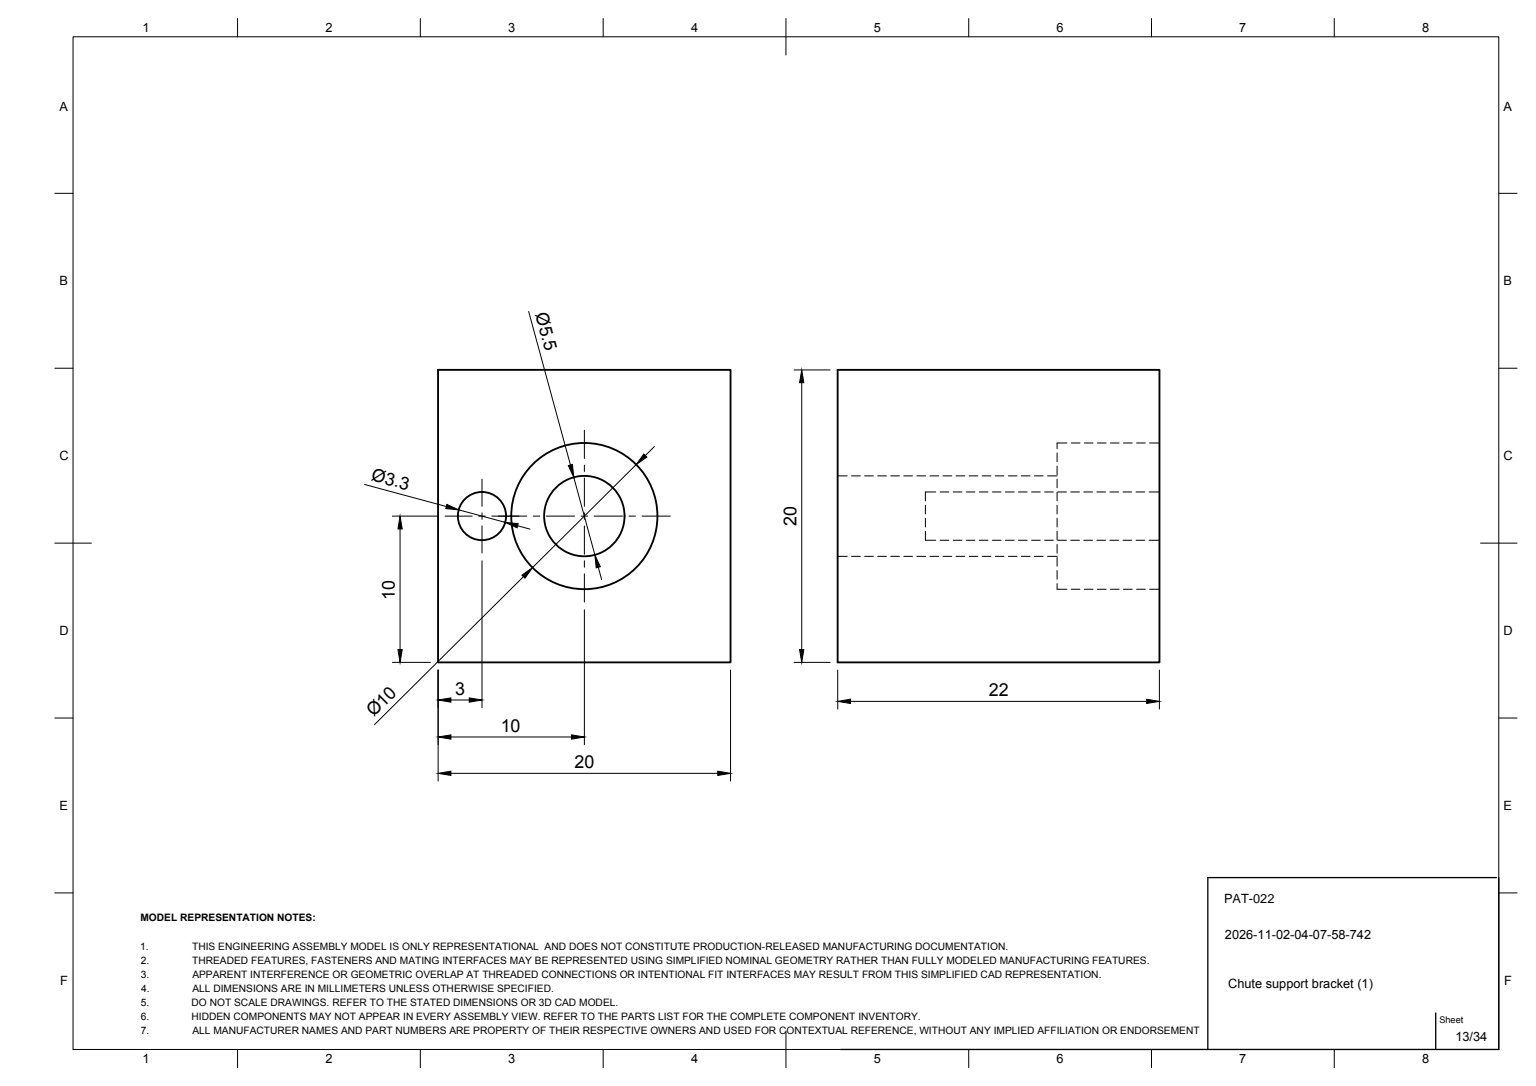
ISO-10303-21;
HEADER;
/* Generated by software containing ST-Developer
 * from STEP Tools, Inc. (www.steptools.com) 
 */

FILE_DESCRIPTION(
/* description */ ('Chute with adjustable gate'),
/* implementation_level */ '2;1');

FILE_NAME(
/* name */ 'Chute support bracket (1).step',
/* time_stamp */ '2026-10-27T10:52:28-07:00',
/* author */ (''),
/* organization */ (''),
/* preprocessor_version */ 'ST-DEVELOPER v20.2',
/* originating_system */ 'Autodesk Translation Framework v15.17.0.0',
/* authorisation */ '');

FILE_SCHEMA (('AUTOMOTIVE_DESIGN { 1 0 10303 214 3 1 1 }'));
ENDSEC;

DATA;
#10=MECHANICAL_DESIGN_GEOMETRIC_PRESENTATION_REPRESENTATION('',(#422),#13094);
#358=SHAPE_REPRESENTATION_RELATIONSHIP('SRR','None',#13259,#390);
#390=ADVANCED_BREP_SHAPE_REPRESENTATION('',(#454),#13068);
#422=STYLED_ITEM('',(#13474),#454);
#454=MANIFOLD_SOLID_BREP('Body1',#7605);
#504=FACE_BOUND('',#1432,.T.);
#505=FACE_BOUND('',#1435,.T.);
#506=FACE_BOUND('',#1438,.T.);
#507=FACE_BOUND('',#1439,.T.);
#644=PLANE('',#8099);
#645=PLANE('',#8103);
#646=PLANE('',#8107);
#647=PLANE('',#8108);
#648=PLANE('',#8109);
#649=PLANE('',#8110);
#650=PLANE('',#8111);
#651=PLANE('',#8112);
#983=FACE_OUTER_BOUND('',#1428,.T.);
#984=FACE_OUTER_BOUND('',#1429,.T.);
#985=FACE_OUTER_BOUND('',#1430,.T.);
#986=FACE_OUTER_BOUND('',#1431,.T.);
#987=FACE_OUTER_BOUND('',#1433,.T.);
#988=FACE_OUTER_BOUND('',#1434,.T.);
#989=FACE_OUTER_BOUND('',#1436,.T.);
#990=FACE_OUTER_BOUND('',#1437,.T.);
#991=FACE_OUTER_BOUND('',#1440,.T.);
#992=FACE_OUTER_BOUND('',#1441,.T.);
#993=FACE_OUTER_BOUND('',#1442,.T.);
#1428=EDGE_LOOP('',(#5492,#5493,#5494,#5495));
#1429=EDGE_LOOP('',(#5496));
#1430=EDGE_LOOP('',(#5497,#5498,#5499,#5500));
#1431=EDGE_LOOP('',(#5501));
#1432=EDGE_LOOP('',(#5502));
#1433=EDGE_LOOP('',(#5503,#5504,#5505,#5506));
#1434=EDGE_LOOP('',(#5507,#5508,#5509,#5510));
#1435=EDGE_LOOP('',(#5511));
#1436=EDGE_LOOP('',(#5512,#5513,#5514,#5515));
#1437=EDGE_LOOP('',(#5516,#5517,#5518,#5519));
#1438=EDGE_LOOP('',(#5520));
#1439=EDGE_LOOP('',(#5521));
#1440=EDGE_LOOP('',(#5522,#5523,#5524,#5525));
#1441=EDGE_LOOP('',(#5526,#5527,#5528,#5529));
#1442=EDGE_LOOP('',(#5530,#5531,#5532,#5533));
#1983=LINE('',#11238,#2760);
#1984=LINE('',#11245,#2761);
#1985=LINE('',#11252,#2762);
#1986=LINE('',#11257,#2763);
#1987=LINE('',#11259,#2764);
#1988=LINE('',#11261,#2765);
#1989=LINE('',#11262,#2766);
#1990=LINE('',#11265,#2767);
#1991=LINE('',#11267,#2768);
#1992=LINE('',#11268,#2769);
#1993=LINE('',#11271,#2770);
#1994=LINE('',#11273,#2771);
#1995=LINE('',#11274,#2772);
#1996=LINE('',#11276,#2773);
#1997=LINE('',#11277,#2774);
#2760=VECTOR('',#9045,0.165);
#2761=VECTOR('',#9054,0.5);
#2762=VECTOR('',#9063,0.275);
#2763=VECTOR('',#9068,1.);
#2764=VECTOR('',#9069,1.);
#2765=VECTOR('',#9070,1.);
#2766=VECTOR('',#9071,1.);
#2767=VECTOR('',#9074,1.);
#2768=VECTOR('',#9075,1.);
#2769=VECTOR('',#9076,1.);
#2770=VECTOR('',#9079,1.);
#2771=VECTOR('',#9080,1.);
#2772=VECTOR('',#9081,1.);
#2773=VECTOR('',#9084,1.);
#2774=VECTOR('',#9085,1.);
#3444=CIRCLE('',#8097,0.165);
#3445=CIRCLE('',#8098,0.165);
#3446=CIRCLE('',#8101,0.5);
#3447=CIRCLE('',#8102,0.5);
#3448=CIRCLE('',#8104,0.275);
#3449=CIRCLE('',#8106,0.275);
#3695=VERTEX_POINT('',#11235);
#3696=VERTEX_POINT('',#11237);
#3697=VERTEX_POINT('',#11242);
#3698=VERTEX_POINT('',#11244);
#3699=VERTEX_POINT('',#11248);
#3700=VERTEX_POINT('',#11251);
#3701=VERTEX_POINT('',#11255);
#3702=VERTEX_POINT('',#11256);
#3703=VERTEX_POINT('',#11258);
#3704=VERTEX_POINT('',#11260);
#3705=VERTEX_POINT('',#11264);
#3706=VERTEX_POINT('',#11266);
#3707=VERTEX_POINT('',#11270);
#3708=VERTEX_POINT('',#11272);
#4379=EDGE_CURVE('',#3695,#3695,#3444,.T.);
#4380=EDGE_CURVE('',#3695,#3696,#1983,.T.);
#4381=EDGE_CURVE('',#3696,#3696,#3445,.T.);
#4382=EDGE_CURVE('',#3697,#3697,#3446,.T.);
#4383=EDGE_CURVE('',#3697,#3698,#1984,.T.);
#4384=EDGE_CURVE('',#3698,#3698,#3447,.T.);
#4385=EDGE_CURVE('',#3699,#3699,#3448,.T.);
#4386=EDGE_CURVE('',#3699,#3700,#1985,.T.);
#4387=EDGE_CURVE('',#3700,#3700,#3449,.T.);
#4388=EDGE_CURVE('',#3701,#3702,#1986,.T.);
#4389=EDGE_CURVE('',#3702,#3703,#1987,.T.);
#4390=EDGE_CURVE('',#3704,#3703,#1988,.T.);
#4391=EDGE_CURVE('',#3701,#3704,#1989,.T.);
#4392=EDGE_CURVE('',#3705,#3701,#1990,.T.);
#4393=EDGE_CURVE('',#3706,#3704,#1991,.T.);
#4394=EDGE_CURVE('',#3705,#3706,#1992,.T.);
#4395=EDGE_CURVE('',#3707,#3705,#1993,.T.);
#4396=EDGE_CURVE('',#3708,#3706,#1994,.T.);
#4397=EDGE_CURVE('',#3707,#3708,#1995,.T.);
#4398=EDGE_CURVE('',#3702,#3707,#1996,.T.);
#4399=EDGE_CURVE('',#3703,#3708,#1997,.T.);
#5492=ORIENTED_EDGE('',*,*,#4379,.F.);
#5493=ORIENTED_EDGE('',*,*,#4380,.T.);
#5494=ORIENTED_EDGE('',*,*,#4381,.T.);
#5495=ORIENTED_EDGE('',*,*,#4380,.F.);
#5496=ORIENTED_EDGE('',*,*,#4381,.F.);
#5497=ORIENTED_EDGE('',*,*,#4382,.F.);
#5498=ORIENTED_EDGE('',*,*,#4383,.T.);
#5499=ORIENTED_EDGE('',*,*,#4384,.T.);
#5500=ORIENTED_EDGE('',*,*,#4383,.F.);
#5501=ORIENTED_EDGE('',*,*,#4384,.F.);
#5502=ORIENTED_EDGE('',*,*,#4385,.F.);
#5503=ORIENTED_EDGE('',*,*,#4385,.T.);
#5504=ORIENTED_EDGE('',*,*,#4386,.T.);
#5505=ORIENTED_EDGE('',*,*,#4387,.F.);
#5506=ORIENTED_EDGE('',*,*,#4386,.F.);
#5507=ORIENTED_EDGE('',*,*,#4388,.T.);
#5508=ORIENTED_EDGE('',*,*,#4389,.T.);
#5509=ORIENTED_EDGE('',*,*,#4390,.F.);
#5510=ORIENTED_EDGE('',*,*,#4391,.F.);
#5511=ORIENTED_EDGE('',*,*,#4387,.T.);
#5512=ORIENTED_EDGE('',*,*,#4392,.T.);
#5513=ORIENTED_EDGE('',*,*,#4391,.T.);
#5514=ORIENTED_EDGE('',*,*,#4393,.F.);
#5515=ORIENTED_EDGE('',*,*,#4394,.F.);
#5516=ORIENTED_EDGE('',*,*,#4395,.T.);
#5517=ORIENTED_EDGE('',*,*,#4394,.T.);
#5518=ORIENTED_EDGE('',*,*,#4396,.F.);
#5519=ORIENTED_EDGE('',*,*,#4397,.F.);
#5520=ORIENTED_EDGE('',*,*,#4379,.T.);
#5521=ORIENTED_EDGE('',*,*,#4382,.T.);
#5522=ORIENTED_EDGE('',*,*,#4398,.T.);
#5523=ORIENTED_EDGE('',*,*,#4397,.T.);
#5524=ORIENTED_EDGE('',*,*,#4399,.F.);
#5525=ORIENTED_EDGE('',*,*,#4389,.F.);
#5526=ORIENTED_EDGE('',*,*,#4399,.T.);
#5527=ORIENTED_EDGE('',*,*,#4396,.T.);
#5528=ORIENTED_EDGE('',*,*,#4393,.T.);
#5529=ORIENTED_EDGE('',*,*,#4390,.T.);
#5530=ORIENTED_EDGE('',*,*,#4398,.F.);
#5531=ORIENTED_EDGE('',*,*,#4388,.F.);
#5532=ORIENTED_EDGE('',*,*,#4392,.F.);
#5533=ORIENTED_EDGE('',*,*,#4395,.F.);
#7121=CYLINDRICAL_SURFACE('',#8096,0.165);
#7122=CYLINDRICAL_SURFACE('',#8100,0.5);
#7123=CYLINDRICAL_SURFACE('',#8105,0.275);
#7251=ADVANCED_FACE('',(#983),#7121,.F.);
#7252=ADVANCED_FACE('',(#984),#644,.F.);
#7253=ADVANCED_FACE('',(#985),#7122,.F.);
#7254=ADVANCED_FACE('',(#986,#504),#645,.F.);
#7255=ADVANCED_FACE('',(#987),#7123,.F.);
#7256=ADVANCED_FACE('',(#988,#505),#646,.T.);
#7257=ADVANCED_FACE('',(#989),#647,.T.);
#7258=ADVANCED_FACE('',(#990,#506,#507),#648,.T.);
#7259=ADVANCED_FACE('',(#991),#649,.T.);
#7260=ADVANCED_FACE('',(#992),#650,.T.);
#7261=ADVANCED_FACE('',(#993),#651,.F.);
#7605=CLOSED_SHELL('',(#7251,#7252,#7253,#7254,#7255,#7256,#7257,#7258,
#7259,#7260,#7261));
#8095=AXIS2_PLACEMENT_3D('',#11233,#9039,#9040);
#8096=AXIS2_PLACEMENT_3D('',#11234,#9041,#9042);
#8097=AXIS2_PLACEMENT_3D('',#11236,#9043,#9044);
#8098=AXIS2_PLACEMENT_3D('',#11239,#9046,#9047);
#8099=AXIS2_PLACEMENT_3D('',#11240,#9048,#9049);
#8100=AXIS2_PLACEMENT_3D('',#11241,#9050,#9051);
#8101=AXIS2_PLACEMENT_3D('',#11243,#9052,#9053);
#8102=AXIS2_PLACEMENT_3D('',#11246,#9055,#9056);
#8103=AXIS2_PLACEMENT_3D('',#11247,#9057,#9058);
#8104=AXIS2_PLACEMENT_3D('',#11249,#9059,#9060);
#8105=AXIS2_PLACEMENT_3D('',#11250,#9061,#9062);
#8106=AXIS2_PLACEMENT_3D('',#11253,#9064,#9065);
#8107=AXIS2_PLACEMENT_3D('',#11254,#9066,#9067);
#8108=AXIS2_PLACEMENT_3D('',#11263,#9072,#9073);
#8109=AXIS2_PLACEMENT_3D('',#11269,#9077,#9078);
#8110=AXIS2_PLACEMENT_3D('',#11275,#9082,#9083);
#8111=AXIS2_PLACEMENT_3D('',#11278,#9086,#9087);
#8112=AXIS2_PLACEMENT_3D('',#11279,#9088,#9089);
#9039=DIRECTION('axis',(0.,0.,1.));
#9040=DIRECTION('refdir',(1.,0.,0.));
#9041=DIRECTION('center_axis',(0.,1.,0.));
#9042=DIRECTION('ref_axis',(1.,0.,0.));
#9043=DIRECTION('center_axis',(0.,1.,0.));
#9044=DIRECTION('ref_axis',(1.,0.,0.));
#9045=DIRECTION('',(0.,1.,0.));
#9046=DIRECTION('center_axis',(0.,1.,0.));
#9047=DIRECTION('ref_axis',(1.,0.,0.));
#9048=DIRECTION('center_axis',(0.,1.,0.));
#9049=DIRECTION('ref_axis',(1.,0.,0.));
#9050=DIRECTION('center_axis',(0.,1.,0.));
#9051=DIRECTION('ref_axis',(1.,0.,0.));
#9052=DIRECTION('center_axis',(0.,1.,0.));
#9053=DIRECTION('ref_axis',(1.,0.,0.));
#9054=DIRECTION('',(0.,1.,0.));
#9055=DIRECTION('center_axis',(0.,1.,0.));
#9056=DIRECTION('ref_axis',(1.,0.,0.));
#9057=DIRECTION('center_axis',(0.,1.,0.));
#9058=DIRECTION('ref_axis',(1.,0.,0.));
#9059=DIRECTION('center_axis',(0.,-1.,0.));
#9060=DIRECTION('ref_axis',(1.,0.,0.));
#9061=DIRECTION('center_axis',(0.,1.,0.));
#9062=DIRECTION('ref_axis',(1.,0.,0.));
#9063=DIRECTION('',(0.,1.,0.));
#9064=DIRECTION('center_axis',(0.,-1.,0.));
#9065=DIRECTION('ref_axis',(1.,0.,0.));
#9066=DIRECTION('center_axis',(0.,1.,0.));
#9067=DIRECTION('ref_axis',(-1.,0.,0.));
#9068=DIRECTION('',(-1.,0.,0.));
#9069=DIRECTION('',(0.,0.,1.));
#9070=DIRECTION('',(-1.,0.,0.));
#9071=DIRECTION('',(0.,0.,1.));
#9072=DIRECTION('center_axis',(1.,0.,0.));
#9073=DIRECTION('ref_axis',(0.,1.,0.));
#9074=DIRECTION('',(0.,1.,0.));
#9075=DIRECTION('',(0.,1.,0.));
#9076=DIRECTION('',(0.,0.,1.));
#9077=DIRECTION('center_axis',(0.,-1.,0.));
#9078=DIRECTION('ref_axis',(1.,0.,0.));
#9079=DIRECTION('',(1.,0.,0.));
#9080=DIRECTION('',(1.,0.,0.));
#9081=DIRECTION('',(0.,0.,1.));
#9082=DIRECTION('center_axis',(-1.,0.,0.));
#9083=DIRECTION('ref_axis',(0.,-1.,0.));
#9084=DIRECTION('',(0.,-1.,0.));
#9085=DIRECTION('',(0.,-1.,0.));
#9086=DIRECTION('center_axis',(0.,0.,1.));
#9087=DIRECTION('ref_axis',(1.,0.,0.));
#9088=DIRECTION('center_axis',(0.,0.,1.));
#9089=DIRECTION('ref_axis',(1.,0.,0.));
#11233=CARTESIAN_POINT('',(0.,0.,0.));
#11234=CARTESIAN_POINT('Origin',(2.3,7.7,7.));
#11235=CARTESIAN_POINT('',(2.135,7.8,7.));
#11236=CARTESIAN_POINT('Origin',(2.3,7.8,7.));
#11237=CARTESIAN_POINT('',(2.135,9.4,7.));
#11238=CARTESIAN_POINT('',(2.135,7.7,7.));
#11239=CARTESIAN_POINT('Origin',(2.3,9.4,7.));
#11240=CARTESIAN_POINT('Origin',(2.3,9.4,7.));
#11241=CARTESIAN_POINT('Origin',(3.,7.7,7.));
#11242=CARTESIAN_POINT('',(2.5,7.8,7.));
#11243=CARTESIAN_POINT('Origin',(3.,7.8,7.));
#11244=CARTESIAN_POINT('',(2.5,8.5,7.));
#11245=CARTESIAN_POINT('',(2.5,7.7,7.));
#11246=CARTESIAN_POINT('Origin',(3.,8.5,7.));
#11247=CARTESIAN_POINT('Origin',(3.,8.5,7.));
#11248=CARTESIAN_POINT('',(2.725,8.5,7.));
#11249=CARTESIAN_POINT('Origin',(3.,8.5,7.));
#11250=CARTESIAN_POINT('Origin',(3.,7.7,7.));
#11251=CARTESIAN_POINT('',(2.725,10.,7.));
#11252=CARTESIAN_POINT('',(2.725,7.7,7.));
#11253=CARTESIAN_POINT('Origin',(3.,10.,7.));
#11254=CARTESIAN_POINT('Origin',(4.,10.,6.));
#11255=CARTESIAN_POINT('',(4.,10.,6.));
#11256=CARTESIAN_POINT('',(2.,10.,6.));
#11257=CARTESIAN_POINT('',(4.,10.,6.));
#11258=CARTESIAN_POINT('',(2.,10.,8.));
#11259=CARTESIAN_POINT('',(2.,10.,6.));
#11260=CARTESIAN_POINT('',(4.,10.,8.));
#11261=CARTESIAN_POINT('',(4.,10.,8.));
#11262=CARTESIAN_POINT('',(4.,10.,6.));
#11263=CARTESIAN_POINT('Origin',(4.,7.8,6.));
#11264=CARTESIAN_POINT('',(4.,7.8,6.));
#11265=CARTESIAN_POINT('',(4.,7.8,6.));
#11266=CARTESIAN_POINT('',(4.,7.8,8.));
#11267=CARTESIAN_POINT('',(4.,7.8,8.));
#11268=CARTESIAN_POINT('',(4.,7.8,6.));
#11269=CARTESIAN_POINT('Origin',(2.,7.8,6.));
#11270=CARTESIAN_POINT('',(2.,7.8,6.));
#11271=CARTESIAN_POINT('',(2.,7.8,6.));
#11272=CARTESIAN_POINT('',(2.,7.8,8.));
#11273=CARTESIAN_POINT('',(2.,7.8,8.));
#11274=CARTESIAN_POINT('',(2.,7.8,6.));
#11275=CARTESIAN_POINT('Origin',(2.,10.,6.));
#11276=CARTESIAN_POINT('',(2.,10.,6.));
#11277=CARTESIAN_POINT('',(2.,10.,8.));
#11278=CARTESIAN_POINT('Origin',(3.,8.9,8.));
#11279=CARTESIAN_POINT('Origin',(3.,8.9,6.));
#13031=UNCERTAINTY_MEASURE_WITH_UNIT(LENGTH_MEASURE(0.001),#13095,
'DISTANCE_ACCURACY_VALUE',
'Maximum model space distance between geometric entities at asserted c
onnectivities');
#13057=UNCERTAINTY_MEASURE_WITH_UNIT(LENGTH_MEASURE(0.001),#13095,
'DISTANCE_ACCURACY_VALUE',
'Maximum model space distance between geometric entities at asserted c
onnectivities');
#13068=(
GEOMETRIC_REPRESENTATION_CONTEXT(3)
GLOBAL_UNCERTAINTY_ASSIGNED_CONTEXT((#13031))
GLOBAL_UNIT_ASSIGNED_CONTEXT((#13095,#13097,#13098))
REPRESENTATION_CONTEXT('','3D')
);
#13094=(
GEOMETRIC_REPRESENTATION_CONTEXT(3)
GLOBAL_UNCERTAINTY_ASSIGNED_CONTEXT((#13057))
GLOBAL_UNIT_ASSIGNED_CONTEXT((#13095,#13097,#13098))
REPRESENTATION_CONTEXT('','3D')
);
#13095=(
LENGTH_UNIT()
NAMED_UNIT(*)
SI_UNIT(.CENTI.,.METRE.)
);
#13097=(
NAMED_UNIT(*)
PLANE_ANGLE_UNIT()
SI_UNIT($,.RADIAN.)
);
#13098=(
NAMED_UNIT(*)
SI_UNIT($,.STERADIAN.)
SOLID_ANGLE_UNIT()
);
#13109=SHAPE_DEFINITION_REPRESENTATION(#13145,#13259);
#13145=PRODUCT_DEFINITION_SHAPE('',$,#13296);
#13259=SHAPE_REPRESENTATION('',(#8095),#13068);
#13285=PRODUCT_DEFINITION_CONTEXT('part definition',#13395,'design');
#13296=PRODUCT_DEFINITION('Chute support bracket (1)',
'Chute support bracket (1)',#13332,#13285);
#13332=PRODUCT_DEFINITION_FORMATION('',$,#13407);
#13395=APPLICATION_CONTEXT(
'Core Data for Automotive Mechanical Design Process');
#13396=PRODUCT_CONTEXT('part definition',#13395,'mechanical');
#13407=PRODUCT('Chute support bracket (1)','Chute support bracket (1)',
'Chute support bracket (1)',(#13396));
#13468=COLOUR_RGB('Dark Blue',0.08,0.2,0.34);
#13469=FILL_AREA_STYLE_COLOUR('',#13468);
#13470=FILL_AREA_STYLE('',(#13469));
#13471=SURFACE_STYLE_FILL_AREA(#13470);
#13472=SURFACE_SIDE_STYLE('',(#13471));
#13473=SURFACE_STYLE_USAGE(.BOTH.,#13472);
#13474=PRESENTATION_STYLE_ASSIGNMENT((#13473));
ENDSEC;
END-ISO-10303-21;
